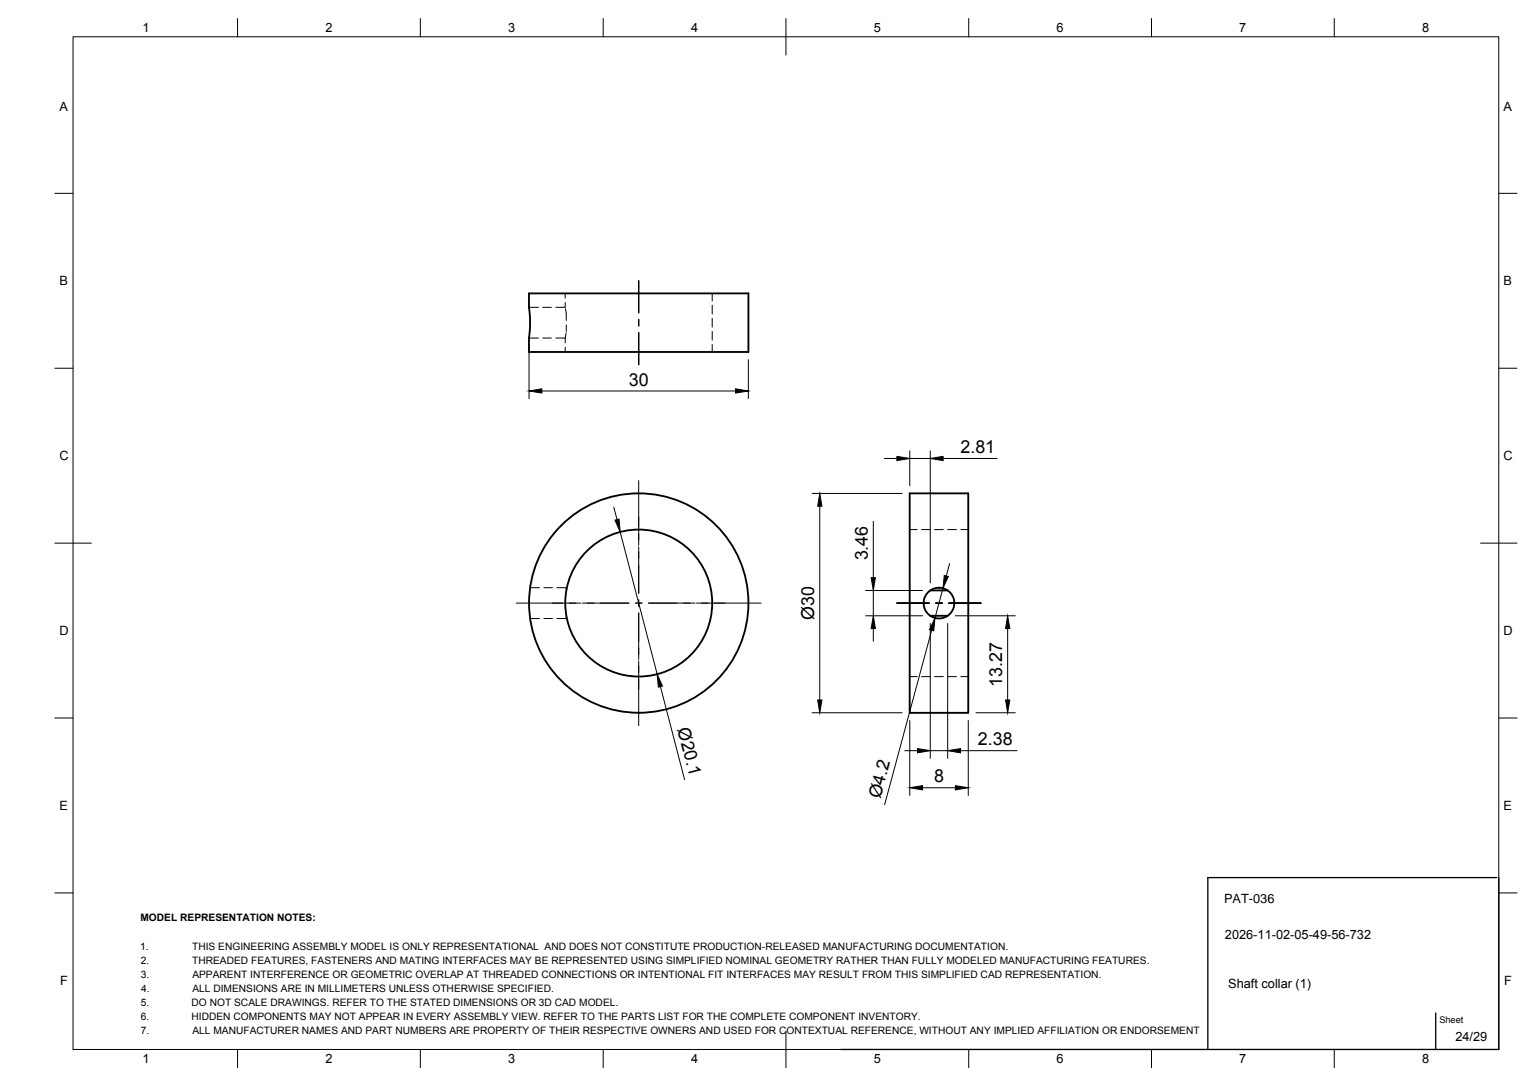
ISO-10303-21;
HEADER;
/* Generated by software containing ST-Developer
 * from STEP Tools, Inc. (www.steptools.com) 
 */

FILE_DESCRIPTION(
/* description */ ('Flange-mounted spindle'),
/* implementation_level */ '2;1');

FILE_NAME(
/* name */ 'Shaft collar (1).step',
/* time_stamp */ '2026-10-27T10:49:51-07:00',
/* author */ (''),
/* organization */ (''),
/* preprocessor_version */ 'ST-DEVELOPER v20.2',
/* originating_system */ 'Autodesk Translation Framework v15.17.0.0',
/* authorisation */ '');

FILE_SCHEMA (('AUTOMOTIVE_DESIGN { 1 0 10303 214 3 1 1 }'));
ENDSEC;

DATA;
#10=MECHANICAL_DESIGN_GEOMETRIC_PRESENTATION_REPRESENTATION('',(#356),#11764);
#239=B_SPLINE_CURVE_WITH_KNOTS('',3,(#10343,#10344,#10345,#10346,#10347,
#10348,#10349,#10350,#10351,#10352,#10353,#10354,#10355,#10356),
 .UNSPECIFIED.,.F.,.F.,(4,2,2,2,2,2,4),(0.756005737987011,0.793568827564647,
0.872922520054201,0.952276212543756,1.03162990503331,1.11098359752287,1.1485466871005),
 .UNSPECIFIED.);
#240=B_SPLINE_CURVE_WITH_KNOTS('',3,(#10362,#10363,#10364,#10365,#10366,
#10367,#10368,#10369,#10370,#10371,#10372,#10373,#10374,#10375,#10376,#10377,
#10378,#10379),.UNSPECIFIED.,.F.,.F.,(4,2,2,2,2,2,2,2,4),(0.,0.079216580773363,
0.158433161546726,0.23764869707457,0.316864232602414,0.396079768130259,
0.475295303658103,0.554511884431466,0.633728465204829),.UNSPECIFIED.);
#241=B_SPLINE_CURVE_WITH_KNOTS('',3,(#10380,#10381,#10382,#10383,#10384,
#10385,#10386,#10387,#10388,#10389,#10390,#10391,#10392,#10393,#10394,#10395,
#10396,#10397),.UNSPECIFIED.,.F.,.F.,(4,2,2,2,2,2,2,2,4),(0.633728465204829,
0.712945045978192,0.792161626751555,0.871377162279399,0.950592697807243,
1.02980823333509,1.10902376886293,1.18824034963629,1.26745693040966),
 .UNSPECIFIED.);
#242=B_SPLINE_CURVE_WITH_KNOTS('',3,(#10400,#10401,#10402,#10403,#10404,
#10405,#10406,#10407,#10408,#10409,#10410,#10411,#10412,#10413),
 .UNSPECIFIED.,.F.,.F.,(4,2,2,2,2,2,4),(0.121154929624506,0.158718019202143,
0.238071711691697,0.317425404181252,0.396779096670807,0.476132789160362,
0.513695878737998),.UNSPECIFIED.);
#301=SHAPE_REPRESENTATION_RELATIONSHIP('SRR','None',#11899,#328);
#328=ADVANCED_BREP_SHAPE_REPRESENTATION('',(#382),#11754);
#356=STYLED_ITEM('',(#12099),#382);
#382=MANIFOLD_SOLID_BREP('Body1',#6150);
#467=FACE_BOUND('',#1258,.T.);
#468=FACE_BOUND('',#1260,.T.);
#469=FACE_BOUND('',#1262,.T.);
#470=FACE_BOUND('',#1264,.T.);
#604=PLANE('',#6750);
#605=PLANE('',#6755);
#606=PLANE('',#6762);
#607=PLANE('',#6763);
#833=FACE_OUTER_BOUND('',#1254,.T.);
#834=FACE_OUTER_BOUND('',#1255,.T.);
#835=FACE_OUTER_BOUND('',#1256,.T.);
#836=FACE_OUTER_BOUND('',#1257,.T.);
#837=FACE_OUTER_BOUND('',#1259,.T.);
#838=FACE_OUTER_BOUND('',#1261,.T.);
#839=FACE_OUTER_BOUND('',#1263,.T.);
#1254=EDGE_LOOP('',(#4667,#4668));
#1255=EDGE_LOOP('',(#4669,#4670,#4671,#4672,#4673,#4674,#4675,#4676,#4677));
#1256=EDGE_LOOP('',(#4678,#4679,#4680));
#1257=EDGE_LOOP('',(#4681,#4682,#4683,#4684));
#1258=EDGE_LOOP('',(#4685,#4686,#4687,#4688));
#1259=EDGE_LOOP('',(#4689,#4690,#4691,#4692));
#1260=EDGE_LOOP('',(#4693,#4694));
#1261=EDGE_LOOP('',(#4695));
#1262=EDGE_LOOP('',(#4696));
#1263=EDGE_LOOP('',(#4697));
#1264=EDGE_LOOP('',(#4698));
#1674=LINE('',#10339,#2096);
#1675=LINE('',#10360,#2097);
#1676=LINE('',#10415,#2098);
#1677=LINE('',#10420,#2099);
#1678=LINE('',#10426,#2100);
#2096=VECTOR('',#7987,1.);
#2097=VECTOR('',#7994,0.21);
#2098=VECTOR('',#7999,1.);
#2099=VECTOR('',#8004,1.005);
#2100=VECTOR('',#8011,1.5);
#2431=CIRCLE('',#6751,0.21);
#2432=CIRCLE('',#6753,0.21);
#2433=CIRCLE('',#6754,0.21);
#2434=CIRCLE('',#6757,1.005);
#2435=CIRCLE('',#6758,1.005);
#2436=CIRCLE('',#6760,1.5);
#2437=CIRCLE('',#6761,1.5);
#2875=VERTEX_POINT('',#10337);
#2876=VERTEX_POINT('',#10338);
#2877=VERTEX_POINT('',#10342);
#2878=VERTEX_POINT('',#10357);
#2879=VERTEX_POINT('',#10359);
#2880=VERTEX_POINT('',#10361);
#2881=VERTEX_POINT('',#10398);
#2882=VERTEX_POINT('',#10417);
#2883=VERTEX_POINT('',#10419);
#2884=VERTEX_POINT('',#10423);
#2885=VERTEX_POINT('',#10425);
#3526=EDGE_CURVE('',#2875,#2876,#1674,.T.);
#3527=EDGE_CURVE('',#2875,#2876,#2431,.T.);
#3528=EDGE_CURVE('',#2877,#2875,#239,.T.);
#3529=EDGE_CURVE('',#2878,#2877,#2432,.T.);
#3530=EDGE_CURVE('',#2878,#2879,#1675,.T.);
#3531=EDGE_CURVE('',#2880,#2879,#240,.T.);
#3532=EDGE_CURVE('',#2879,#2880,#241,.T.);
#3533=EDGE_CURVE('',#2881,#2878,#2433,.T.);
#3534=EDGE_CURVE('',#2876,#2881,#242,.T.);
#3535=EDGE_CURVE('',#2881,#2877,#1676,.T.);
#3536=EDGE_CURVE('',#2882,#2882,#2434,.T.);
#3537=EDGE_CURVE('',#2882,#2883,#1677,.T.);
#3538=EDGE_CURVE('',#2883,#2883,#2435,.T.);
#3539=EDGE_CURVE('',#2884,#2884,#2436,.T.);
#3540=EDGE_CURVE('',#2884,#2885,#1678,.T.);
#3541=EDGE_CURVE('',#2885,#2885,#2437,.T.);
#4667=ORIENTED_EDGE('',*,*,#3526,.F.);
#4668=ORIENTED_EDGE('',*,*,#3527,.T.);
#4669=ORIENTED_EDGE('',*,*,#3528,.F.);
#4670=ORIENTED_EDGE('',*,*,#3529,.F.);
#4671=ORIENTED_EDGE('',*,*,#3530,.T.);
#4672=ORIENTED_EDGE('',*,*,#3531,.F.);
#4673=ORIENTED_EDGE('',*,*,#3532,.F.);
#4674=ORIENTED_EDGE('',*,*,#3530,.F.);
#4675=ORIENTED_EDGE('',*,*,#3533,.F.);
#4676=ORIENTED_EDGE('',*,*,#3534,.F.);
#4677=ORIENTED_EDGE('',*,*,#3527,.F.);
#4678=ORIENTED_EDGE('',*,*,#3535,.F.);
#4679=ORIENTED_EDGE('',*,*,#3533,.T.);
#4680=ORIENTED_EDGE('',*,*,#3529,.T.);
#4681=ORIENTED_EDGE('',*,*,#3536,.F.);
#4682=ORIENTED_EDGE('',*,*,#3537,.T.);
#4683=ORIENTED_EDGE('',*,*,#3538,.T.);
#4684=ORIENTED_EDGE('',*,*,#3537,.F.);
#4685=ORIENTED_EDGE('',*,*,#3534,.T.);
#4686=ORIENTED_EDGE('',*,*,#3535,.T.);
#4687=ORIENTED_EDGE('',*,*,#3528,.T.);
#4688=ORIENTED_EDGE('',*,*,#3526,.T.);
#4689=ORIENTED_EDGE('',*,*,#3539,.F.);
#4690=ORIENTED_EDGE('',*,*,#3540,.T.);
#4691=ORIENTED_EDGE('',*,*,#3541,.T.);
#4692=ORIENTED_EDGE('',*,*,#3540,.F.);
#4693=ORIENTED_EDGE('',*,*,#3531,.T.);
#4694=ORIENTED_EDGE('',*,*,#3532,.T.);
#4695=ORIENTED_EDGE('',*,*,#3539,.T.);
#4696=ORIENTED_EDGE('',*,*,#3536,.T.);
#4697=ORIENTED_EDGE('',*,*,#3541,.F.);
#4698=ORIENTED_EDGE('',*,*,#3538,.F.);
#5677=CYLINDRICAL_SURFACE('',#6752,0.21);
#5678=CYLINDRICAL_SURFACE('',#6756,1.005);
#5679=CYLINDRICAL_SURFACE('',#6759,1.5);
#5944=ADVANCED_FACE('',(#833),#604,.T.);
#5945=ADVANCED_FACE('',(#834),#5677,.F.);
#5946=ADVANCED_FACE('',(#835),#605,.T.);
#5947=ADVANCED_FACE('',(#836,#467),#5678,.F.);
#5948=ADVANCED_FACE('',(#837,#468),#5679,.T.);
#5949=ADVANCED_FACE('',(#838,#469),#606,.T.);
#5950=ADVANCED_FACE('',(#839,#470),#607,.F.);
#6150=CLOSED_SHELL('',(#5944,#5945,#5946,#5947,#5948,#5949,#5950));
#6749=AXIS2_PLACEMENT_3D('',#10335,#7983,#7984);
#6750=AXIS2_PLACEMENT_3D('',#10336,#7985,#7986);
#6751=AXIS2_PLACEMENT_3D('',#10340,#7988,#7989);
#6752=AXIS2_PLACEMENT_3D('',#10341,#7990,#7991);
#6753=AXIS2_PLACEMENT_3D('',#10358,#7992,#7993);
#6754=AXIS2_PLACEMENT_3D('',#10399,#7995,#7996);
#6755=AXIS2_PLACEMENT_3D('',#10414,#7997,#7998);
#6756=AXIS2_PLACEMENT_3D('',#10416,#8000,#8001);
#6757=AXIS2_PLACEMENT_3D('',#10418,#8002,#8003);
#6758=AXIS2_PLACEMENT_3D('',#10421,#8005,#8006);
#6759=AXIS2_PLACEMENT_3D('',#10422,#8007,#8008);
#6760=AXIS2_PLACEMENT_3D('',#10424,#8009,#8010);
#6761=AXIS2_PLACEMENT_3D('',#10427,#8012,#8013);
#6762=AXIS2_PLACEMENT_3D('',#10428,#8014,#8015);
#6763=AXIS2_PLACEMENT_3D('',#10429,#8016,#8017);
#7983=DIRECTION('axis',(0.,0.,1.));
#7984=DIRECTION('refdir',(1.,0.,0.));
#7985=DIRECTION('center_axis',(0.,0.,1.));
#7986=DIRECTION('ref_axis',(1.,0.,0.));
#7987=DIRECTION('',(0.,1.,0.));
#7988=DIRECTION('center_axis',(0.,0.,1.));
#7989=DIRECTION('ref_axis',(1.,0.,0.));
#7990=DIRECTION('center_axis',(0.,0.,1.));
#7991=DIRECTION('ref_axis',(1.,0.,0.));
#7992=DIRECTION('center_axis',(0.,0.,1.));
#7993=DIRECTION('ref_axis',(1.,0.,0.));
#7994=DIRECTION('',(0.,0.,1.));
#7995=DIRECTION('center_axis',(0.,0.,1.));
#7996=DIRECTION('ref_axis',(1.,0.,0.));
#7997=DIRECTION('center_axis',(0.,0.,1.));
#7998=DIRECTION('ref_axis',(1.,0.,0.));
#7999=DIRECTION('',(0.,-1.,0.));
#8000=DIRECTION('center_axis',(0.,1.,0.));
#8001=DIRECTION('ref_axis',(1.,0.,0.));
#8002=DIRECTION('center_axis',(0.,-1.,0.));
#8003=DIRECTION('ref_axis',(1.,0.,0.));
#8004=DIRECTION('',(0.,-1.,0.));
#8005=DIRECTION('center_axis',(0.,-1.,0.));
#8006=DIRECTION('ref_axis',(1.,0.,0.));
#8007=DIRECTION('center_axis',(0.,1.,0.));
#8008=DIRECTION('ref_axis',(1.,0.,0.));
#8009=DIRECTION('center_axis',(0.,1.,0.));
#8010=DIRECTION('ref_axis',(1.,0.,0.));
#8011=DIRECTION('',(0.,-1.,0.));
#8012=DIRECTION('center_axis',(0.,1.,0.));
#8013=DIRECTION('ref_axis',(1.,0.,0.));
#8014=DIRECTION('center_axis',(0.,1.,0.));
#8015=DIRECTION('ref_axis',(1.,0.,0.));
#8016=DIRECTION('center_axis',(0.,1.,0.));
#8017=DIRECTION('ref_axis',(1.,0.,0.));
#10335=CARTESIAN_POINT('',(0.,0.,0.));
#10336=CARTESIAN_POINT('Origin',(0.,2.85,8.99));
#10337=CARTESIAN_POINT('',(0.172988438920061,2.73094119100209,8.99));
#10338=CARTESIAN_POINT('',(0.172988438920061,2.96905880899791,8.99));
#10339=CARTESIAN_POINT('',(0.172988438920061,2.45,8.99));
#10340=CARTESIAN_POINT('Origin',(0.,2.85,8.99));
#10341=CARTESIAN_POINT('Origin',(0.,2.85,8.99));
#10342=CARTESIAN_POINT('',(-0.172988438920061,2.73094119100209,8.99));
#10343=CARTESIAN_POINT('Ctrl Pts',(-0.172988438920061,2.73094119100209,
8.99));
#10344=CARTESIAN_POINT('Ctrl Pts',(-0.165594865311318,2.72019857760471,
8.99129192197638));
#10345=CARTESIAN_POINT('Ctrl Pts',(-0.157297138725608,2.71031229062726,
8.99265394943905));
#10346=CARTESIAN_POINT('Ctrl Pts',(-0.129892073845076,2.68290722574673,
8.9967480843909));
#10347=CARTESIAN_POINT('Ctrl Pts',(-0.106330167759285,2.66675794366705,
8.99969589327638));
#10348=CARTESIAN_POINT('Ctrl Pts',(-0.0546129046324105,2.64530220603509,
9.00385029472357));
#10349=CARTESIAN_POINT('Ctrl Pts',(-0.0264512308298517,2.64,9.005));
#10350=CARTESIAN_POINT('Ctrl Pts',(0.0264512308298516,2.64,9.005));
#10351=CARTESIAN_POINT('Ctrl Pts',(0.0546129046324104,2.64530220603509,
9.00385029472357));
#10352=CARTESIAN_POINT('Ctrl Pts',(0.106330167759284,2.66675794366705,8.99969589327638));
#10353=CARTESIAN_POINT('Ctrl Pts',(0.129892073845076,2.68290722574673,8.9967480843909));
#10354=CARTESIAN_POINT('Ctrl Pts',(0.157297138725608,2.71031229062726,8.99265394943905));
#10355=CARTESIAN_POINT('Ctrl Pts',(0.165594865311318,2.72019857760471,8.99129192197638));
#10356=CARTESIAN_POINT('Ctrl Pts',(0.172988438920061,2.73094119100209,8.99));
#10357=CARTESIAN_POINT('',(-0.21,2.85,8.99));
#10358=CARTESIAN_POINT('Origin',(0.,2.85,8.99));
#10359=CARTESIAN_POINT('',(-0.21,2.85,9.48522725533839));
#10360=CARTESIAN_POINT('',(-0.21,2.85,8.99));
#10361=CARTESIAN_POINT('',(0.21,2.85,9.48522725533839));
#10362=CARTESIAN_POINT('Ctrl Pts',(0.21,2.85,9.48522725533839));
#10363=CARTESIAN_POINT('Ctrl Pts',(0.21,2.82359447307555,9.48522725533839));
#10364=CARTESIAN_POINT('Ctrl Pts',(0.204715737269596,2.79545292590929,9.48600415954412));
#10365=CARTESIAN_POINT('Ctrl Pts',(0.183273763036332,2.74372373109487,9.48880073282317));
#10366=CARTESIAN_POINT('Ctrl Pts',(0.167117923970394,2.72013307587204,9.49077897157582));
#10367=CARTESIAN_POINT('Ctrl Pts',(0.129867169887369,2.68288232178902,9.49448481141327));
#10368=CARTESIAN_POINT('Ctrl Pts',(0.106276408305765,2.66672628999865,9.49645455657129));
#10369=CARTESIAN_POINT('Ctrl Pts',(0.0545468514059001,2.64528417517378,
9.49923165515646));
#10370=CARTESIAN_POINT('Ctrl Pts',(0.0264051785092814,2.64,9.5));
#10371=CARTESIAN_POINT('Ctrl Pts',(-0.0264051785092814,2.64,9.5));
#10372=CARTESIAN_POINT('Ctrl Pts',(-0.0545468514059001,2.64528417517378,
9.49923165515646));
#10373=CARTESIAN_POINT('Ctrl Pts',(-0.106276408305765,2.66672628999865,
9.49645455657129));
#10374=CARTESIAN_POINT('Ctrl Pts',(-0.129867169887369,2.68288232178902,
9.49448481141327));
#10375=CARTESIAN_POINT('Ctrl Pts',(-0.167117923970394,2.72013307587204,
9.49077897157582));
#10376=CARTESIAN_POINT('Ctrl Pts',(-0.183273763036332,2.74372373109487,
9.48880073282317));
#10377=CARTESIAN_POINT('Ctrl Pts',(-0.204715737269596,2.79545292590929,
9.48600415954412));
#10378=CARTESIAN_POINT('Ctrl Pts',(-0.21,2.82359447307555,9.48522725533839));
#10379=CARTESIAN_POINT('Ctrl Pts',(-0.21,2.85,9.48522725533839));
#10380=CARTESIAN_POINT('Ctrl Pts',(-0.21,2.85,9.48522725533839));
#10381=CARTESIAN_POINT('Ctrl Pts',(-0.21,2.87640552692445,9.48522725533839));
#10382=CARTESIAN_POINT('Ctrl Pts',(-0.204715737269596,2.90454707409071,
9.48600415954412));
#10383=CARTESIAN_POINT('Ctrl Pts',(-0.183273763036332,2.95627626890513,
9.48880073282317));
#10384=CARTESIAN_POINT('Ctrl Pts',(-0.167117923970394,2.97986692412796,
9.49077897157582));
#10385=CARTESIAN_POINT('Ctrl Pts',(-0.129867169887369,3.01711767821098,
9.49448481141327));
#10386=CARTESIAN_POINT('Ctrl Pts',(-0.106276408305765,3.03327371000135,
9.49645455657129));
#10387=CARTESIAN_POINT('Ctrl Pts',(-0.0545468514059001,3.05471582482622,
9.49923165515646));
#10388=CARTESIAN_POINT('Ctrl Pts',(-0.0264051785092814,3.06,9.5));
#10389=CARTESIAN_POINT('Ctrl Pts',(0.0264051785092814,3.06,9.5));
#10390=CARTESIAN_POINT('Ctrl Pts',(0.0545468514059005,3.05471582482622,
9.49923165515645));
#10391=CARTESIAN_POINT('Ctrl Pts',(0.106276408305765,3.03327371000135,9.49645455657129));
#10392=CARTESIAN_POINT('Ctrl Pts',(0.129867169887369,3.01711767821098,9.49448481141327));
#10393=CARTESIAN_POINT('Ctrl Pts',(0.167117923970394,2.97986692412796,9.49077897157582));
#10394=CARTESIAN_POINT('Ctrl Pts',(0.183273763036332,2.95627626890513,9.48880073282317));
#10395=CARTESIAN_POINT('Ctrl Pts',(0.204715737269596,2.90454707409071,9.48600415954412));
#10396=CARTESIAN_POINT('Ctrl Pts',(0.21,2.87640552692445,9.48522725533839));
#10397=CARTESIAN_POINT('Ctrl Pts',(0.21,2.85,9.48522725533839));
#10398=CARTESIAN_POINT('',(-0.172988438920061,2.96905880899791,8.99));
#10399=CARTESIAN_POINT('Origin',(0.,2.85,8.99));
#10400=CARTESIAN_POINT('Ctrl Pts',(0.172988438920061,2.96905880899791,8.99));
#10401=CARTESIAN_POINT('Ctrl Pts',(0.165594865311318,2.97980142239529,8.99129192197638));
#10402=CARTESIAN_POINT('Ctrl Pts',(0.157297138725609,2.98968770937274,8.99265394943905));
#10403=CARTESIAN_POINT('Ctrl Pts',(0.129892073845076,3.01709277425327,8.9967480843909));
#10404=CARTESIAN_POINT('Ctrl Pts',(0.106330167759284,3.03324205633295,8.99969589327638));
#10405=CARTESIAN_POINT('Ctrl Pts',(0.0546129046324105,3.05469779396491,
9.00385029472357));
#10406=CARTESIAN_POINT('Ctrl Pts',(0.0264512308298516,3.06,9.005));
#10407=CARTESIAN_POINT('Ctrl Pts',(-0.0264512308298516,3.06,9.005));
#10408=CARTESIAN_POINT('Ctrl Pts',(-0.0546129046324104,3.05469779396491,
9.00385029472357));
#10409=CARTESIAN_POINT('Ctrl Pts',(-0.106330167759284,3.03324205633295,
8.99969589327638));
#10410=CARTESIAN_POINT('Ctrl Pts',(-0.129892073845076,3.01709277425327,
8.9967480843909));
#10411=CARTESIAN_POINT('Ctrl Pts',(-0.157297138725609,2.98968770937274,
8.99265394943905));
#10412=CARTESIAN_POINT('Ctrl Pts',(-0.165594865311319,2.97980142239529,
8.99129192197638));
#10413=CARTESIAN_POINT('Ctrl Pts',(-0.172988438920062,2.96905880899791,
8.99));
#10414=CARTESIAN_POINT('Origin',(0.,2.85,8.99));
#10415=CARTESIAN_POINT('',(-0.172988438920061,2.45,8.99));
#10416=CARTESIAN_POINT('Origin',(0.,2.45,8.));
#10417=CARTESIAN_POINT('',(-1.005,3.25,8.));
#10418=CARTESIAN_POINT('Origin',(0.,3.25,8.));
#10419=CARTESIAN_POINT('',(-1.005,2.45,8.));
#10420=CARTESIAN_POINT('',(-1.005,2.45,8.));
#10421=CARTESIAN_POINT('Origin',(0.,2.45,8.));
#10422=CARTESIAN_POINT('Origin',(0.,2.45,8.));
#10423=CARTESIAN_POINT('',(-1.5,3.25,8.));
#10424=CARTESIAN_POINT('Origin',(0.,3.25,8.));
#10425=CARTESIAN_POINT('',(-1.5,2.45,8.));
#10426=CARTESIAN_POINT('',(-1.5,2.45,8.));
#10427=CARTESIAN_POINT('Origin',(0.,2.45,8.));
#10428=CARTESIAN_POINT('Origin',(0.,3.25,8.));
#10429=CARTESIAN_POINT('Origin',(0.,2.45,8.));
#11722=UNCERTAINTY_MEASURE_WITH_UNIT(LENGTH_MEASURE(0.001),#11765,
'DISTANCE_ACCURACY_VALUE',
'Maximum model space distance between geometric entities at asserted c
onnectivities');
#11732=UNCERTAINTY_MEASURE_WITH_UNIT(LENGTH_MEASURE(0.001),#11765,
'DISTANCE_ACCURACY_VALUE',
'Maximum model space distance between geometric entities at asserted c
onnectivities');
#11754=(
GEOMETRIC_REPRESENTATION_CONTEXT(3)
GLOBAL_UNCERTAINTY_ASSIGNED_CONTEXT((#11722))
GLOBAL_UNIT_ASSIGNED_CONTEXT((#11765,#11767,#11768))
REPRESENTATION_CONTEXT('','3D')
);
#11764=(
GEOMETRIC_REPRESENTATION_CONTEXT(3)
GLOBAL_UNCERTAINTY_ASSIGNED_CONTEXT((#11732))
GLOBAL_UNIT_ASSIGNED_CONTEXT((#11765,#11767,#11768))
REPRESENTATION_CONTEXT('','3D')
);
#11765=(
LENGTH_UNIT()
NAMED_UNIT(*)
SI_UNIT(.CENTI.,.METRE.)
);
#11767=(
NAMED_UNIT(*)
PLANE_ANGLE_UNIT()
SI_UNIT($,.RADIAN.)
);
#11768=(
NAMED_UNIT(*)
SI_UNIT($,.STERADIAN.)
SOLID_ANGLE_UNIT()
);
#11790=SHAPE_DEFINITION_REPRESENTATION(#11823,#11899);
#11823=PRODUCT_DEFINITION_SHAPE('',$,#11931);
#11899=SHAPE_REPRESENTATION('',(#6749),#11754);
#11909=PRODUCT_DEFINITION_CONTEXT('part definition',#12004,'design');
#11931=PRODUCT_DEFINITION('Shaft collar (1)','Shaft collar (1)',#11962,#11909);
#11962=PRODUCT_DEFINITION_FORMATION('',$,#12027);
#12004=APPLICATION_CONTEXT(
'Core Data for Automotive Mechanical Design Process');
#12005=PRODUCT_CONTEXT('part definition',#12004,'mechanical');
#12027=PRODUCT('Shaft collar (1)','Shaft collar (1)','Shaft collar (1)',(#12005));
#12093=COLOUR_RGB('Grey',0.48,0.52,0.57);
#12094=FILL_AREA_STYLE_COLOUR('',#12093);
#12095=FILL_AREA_STYLE('',(#12094));
#12096=SURFACE_STYLE_FILL_AREA(#12095);
#12097=SURFACE_SIDE_STYLE('',(#12096));
#12098=SURFACE_STYLE_USAGE(.BOTH.,#12097);
#12099=PRESENTATION_STYLE_ASSIGNMENT((#12098));
ENDSEC;
END-ISO-10303-21;
